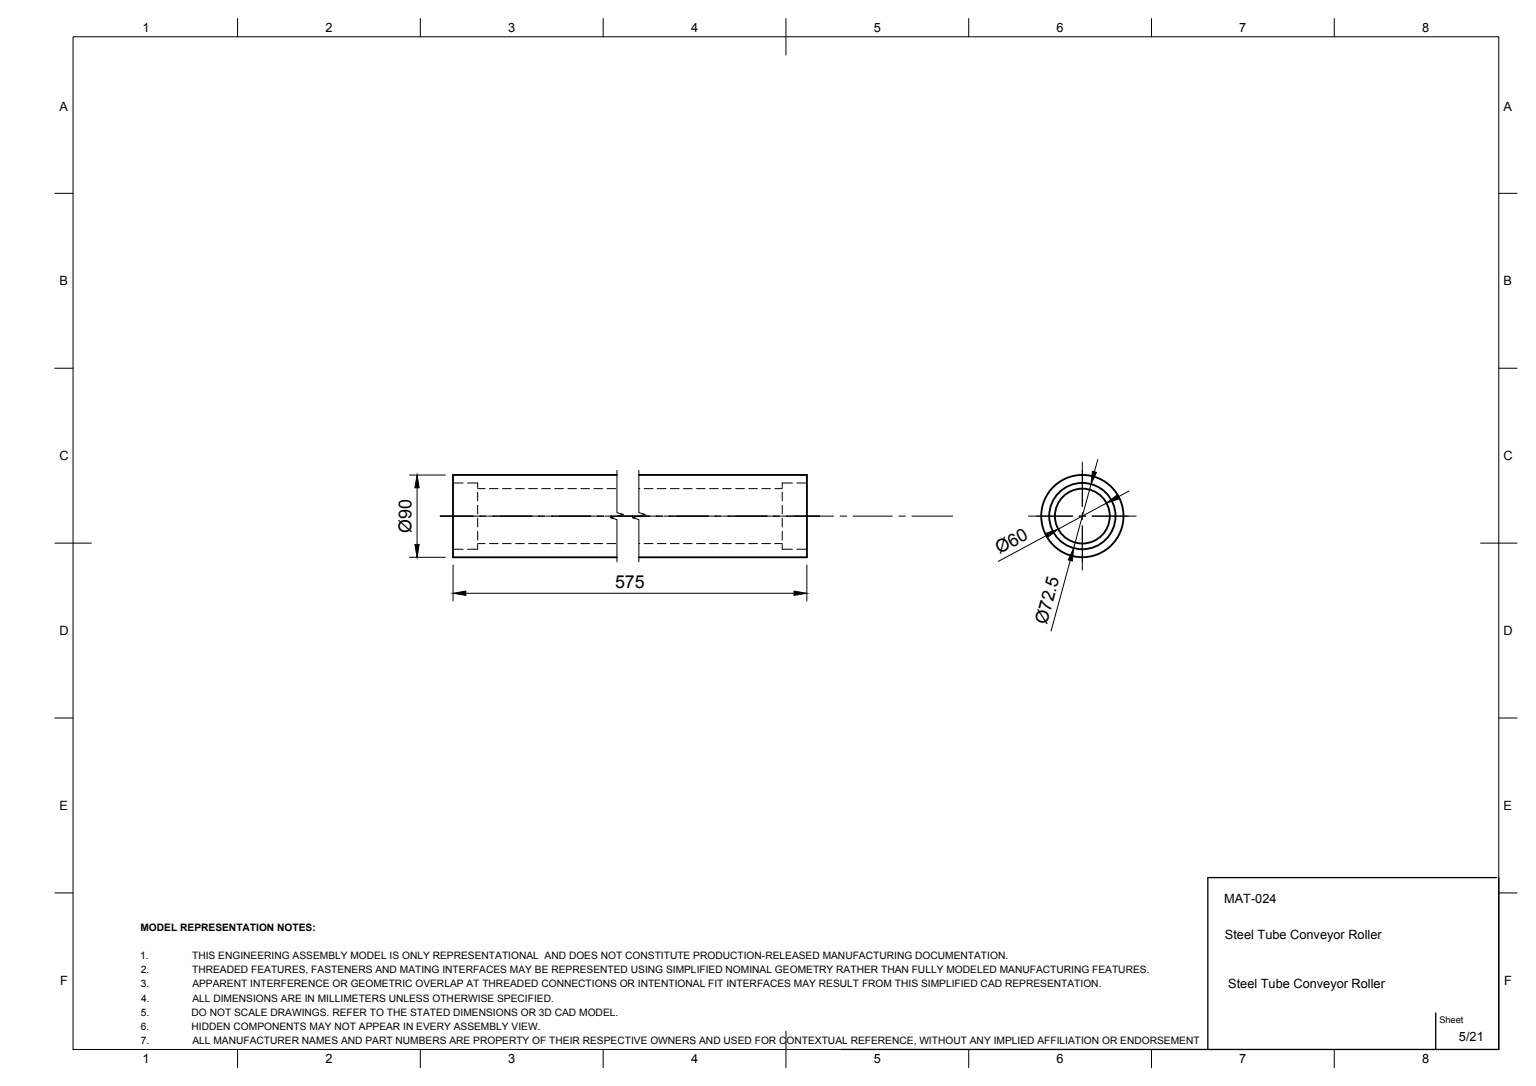
ISO-10303-21;
HEADER;
/* Generated by software containing ST-Developer
 * from STEP Tools, Inc. (www.steptools.com) 
 */

FILE_DESCRIPTION(
/* description */ ('STEP AP214'),
/* implementation_level */ '2;1');

FILE_NAME(
/* name */ 'Steel Tube Conveyor Roller.step',
/* time_stamp */ '2026-11-14T06:34:07-08:00',
/* author */ (''),
/* organization */ (''),
/* preprocessor_version */ 'ST-DEVELOPER v20.2',
/* originating_system */ 'Autodesk Translation Framework v15.17.0.0',
/* authorisation */ '');

FILE_SCHEMA (('AUTOMOTIVE_DESIGN { 1 0 10303 214 3 1 1 }'));
ENDSEC;

DATA;
#10=MECHANICAL_DESIGN_GEOMETRIC_PRESENTATION_REPRESENTATION('',(#7286),#310623);
#7229=SHAPE_REPRESENTATION_RELATIONSHIP('SRR','None',#310902,#7246);
#7246=ADVANCED_BREP_SHAPE_REPRESENTATION('',(#7354),#310611);
#7286=STYLED_ITEM('',(#311003),#7354);
#7354=MANIFOLD_SOLID_BREP('Body1',#93736);
#7638=FACE_BOUND('',#19943,.T.);
#7639=FACE_BOUND('',#19945,.T.);
#7640=FACE_BOUND('',#19947,.T.);
#7641=FACE_BOUND('',#19949,.T.);
#8549=PLANE('',#104125);
#8550=PLANE('',#104126);
#8551=PLANE('',#104127);
#8552=PLANE('',#104128);
#13952=FACE_OUTER_BOUND('',#19938,.T.);
#13953=FACE_OUTER_BOUND('',#19939,.T.);
#13954=FACE_OUTER_BOUND('',#19940,.T.);
#13955=FACE_OUTER_BOUND('',#19941,.T.);
#13956=FACE_OUTER_BOUND('',#19942,.T.);
#13957=FACE_OUTER_BOUND('',#19944,.T.);
#13958=FACE_OUTER_BOUND('',#19946,.T.);
#13959=FACE_OUTER_BOUND('',#19948,.T.);
#19938=EDGE_LOOP('',(#83519,#83520,#83521,#83522));
#19939=EDGE_LOOP('',(#83523,#83524,#83525,#83526));
#19940=EDGE_LOOP('',(#83527,#83528,#83529,#83530));
#19941=EDGE_LOOP('',(#83531,#83532,#83533,#83534));
#19942=EDGE_LOOP('',(#83535));
#19943=EDGE_LOOP('',(#83536));
#19944=EDGE_LOOP('',(#83537));
#19945=EDGE_LOOP('',(#83538));
#19946=EDGE_LOOP('',(#83539));
#19947=EDGE_LOOP('',(#83540));
#19948=EDGE_LOOP('',(#83541));
#19949=EDGE_LOOP('',(#83542));
#24431=LINE('',#275301,#28778);
#24432=LINE('',#275307,#28779);
#24433=LINE('',#275313,#28780);
#24434=LINE('',#275319,#28781);
#28778=VECTOR('',#129118,36.25);
#28779=VECTOR('',#129125,36.25);
#28780=VECTOR('',#129132,45.);
#28781=VECTOR('',#129139,30.);
#34879=CIRCLE('',#104114,36.25);
#34880=CIRCLE('',#104115,36.25);
#34881=CIRCLE('',#104117,36.25);
#34882=CIRCLE('',#104118,36.25);
#34883=CIRCLE('',#104120,45.);
#34884=CIRCLE('',#104121,45.);
#34885=CIRCLE('',#104123,30.);
#34886=CIRCLE('',#104124,30.);
#42853=VERTEX_POINT('',#275298);
#42854=VERTEX_POINT('',#275300);
#42855=VERTEX_POINT('',#275304);
#42856=VERTEX_POINT('',#275306);
#42857=VERTEX_POINT('',#275310);
#42858=VERTEX_POINT('',#275312);
#42859=VERTEX_POINT('',#275316);
#42860=VERTEX_POINT('',#275318);
#56539=EDGE_CURVE('',#42853,#42853,#34879,.T.);
#56540=EDGE_CURVE('',#42853,#42854,#24431,.T.);
#56541=EDGE_CURVE('',#42854,#42854,#34880,.T.);
#56542=EDGE_CURVE('',#42855,#42855,#34881,.T.);
#56543=EDGE_CURVE('',#42855,#42856,#24432,.T.);
#56544=EDGE_CURVE('',#42856,#42856,#34882,.T.);
#56545=EDGE_CURVE('',#42857,#42857,#34883,.T.);
#56546=EDGE_CURVE('',#42857,#42858,#24433,.T.);
#56547=EDGE_CURVE('',#42858,#42858,#34884,.T.);
#56548=EDGE_CURVE('',#42859,#42859,#34885,.T.);
#56549=EDGE_CURVE('',#42859,#42860,#24434,.T.);
#56550=EDGE_CURVE('',#42860,#42860,#34886,.T.);
#83519=ORIENTED_EDGE('',*,*,#56539,.T.);
#83520=ORIENTED_EDGE('',*,*,#56540,.T.);
#83521=ORIENTED_EDGE('',*,*,#56541,.F.);
#83522=ORIENTED_EDGE('',*,*,#56540,.F.);
#83523=ORIENTED_EDGE('',*,*,#56542,.F.);
#83524=ORIENTED_EDGE('',*,*,#56543,.T.);
#83525=ORIENTED_EDGE('',*,*,#56544,.T.);
#83526=ORIENTED_EDGE('',*,*,#56543,.F.);
#83527=ORIENTED_EDGE('',*,*,#56545,.T.);
#83528=ORIENTED_EDGE('',*,*,#56546,.T.);
#83529=ORIENTED_EDGE('',*,*,#56547,.F.);
#83530=ORIENTED_EDGE('',*,*,#56546,.F.);
#83531=ORIENTED_EDGE('',*,*,#56548,.T.);
#83532=ORIENTED_EDGE('',*,*,#56549,.T.);
#83533=ORIENTED_EDGE('',*,*,#56550,.T.);
#83534=ORIENTED_EDGE('',*,*,#56549,.F.);
#83535=ORIENTED_EDGE('',*,*,#56547,.T.);
#83536=ORIENTED_EDGE('',*,*,#56544,.F.);
#83537=ORIENTED_EDGE('',*,*,#56545,.F.);
#83538=ORIENTED_EDGE('',*,*,#56541,.T.);
#83539=ORIENTED_EDGE('',*,*,#56542,.T.);
#83540=ORIENTED_EDGE('',*,*,#56548,.F.);
#83541=ORIENTED_EDGE('',*,*,#56539,.F.);
#83542=ORIENTED_EDGE('',*,*,#56550,.F.);
#87775=CYLINDRICAL_SURFACE('',#104113,36.25);
#87776=CYLINDRICAL_SURFACE('',#104116,36.25);
#87777=CYLINDRICAL_SURFACE('',#104119,45.);
#87778=CYLINDRICAL_SURFACE('',#104122,30.);
#93231=ADVANCED_FACE('',(#13952),#87775,.F.);
#93232=ADVANCED_FACE('',(#13953),#87776,.F.);
#93233=ADVANCED_FACE('',(#13954),#87777,.T.);
#93234=ADVANCED_FACE('',(#13955),#87778,.F.);
#93235=ADVANCED_FACE('',(#13956,#7638),#8549,.T.);
#93236=ADVANCED_FACE('',(#13957,#7639),#8550,.F.);
#93237=ADVANCED_FACE('',(#13958,#7640),#8551,.T.);
#93238=ADVANCED_FACE('',(#13959,#7641),#8552,.T.);
#93736=CLOSED_SHELL('',(#93231,#93232,#93233,#93234,#93235,#93236,#93237,
#93238));
#104112=AXIS2_PLACEMENT_3D('',#275296,#129112,#129113);
#104113=AXIS2_PLACEMENT_3D('',#275297,#129114,#129115);
#104114=AXIS2_PLACEMENT_3D('',#275299,#129116,#129117);
#104115=AXIS2_PLACEMENT_3D('',#275302,#129119,#129120);
#104116=AXIS2_PLACEMENT_3D('',#275303,#129121,#129122);
#104117=AXIS2_PLACEMENT_3D('',#275305,#129123,#129124);
#104118=AXIS2_PLACEMENT_3D('',#275308,#129126,#129127);
#104119=AXIS2_PLACEMENT_3D('',#275309,#129128,#129129);
#104120=AXIS2_PLACEMENT_3D('',#275311,#129130,#129131);
#104121=AXIS2_PLACEMENT_3D('',#275314,#129133,#129134);
#104122=AXIS2_PLACEMENT_3D('',#275315,#129135,#129136);
#104123=AXIS2_PLACEMENT_3D('',#275317,#129137,#129138);
#104124=AXIS2_PLACEMENT_3D('',#275320,#129140,#129141);
#104125=AXIS2_PLACEMENT_3D('',#275321,#129142,#129143);
#104126=AXIS2_PLACEMENT_3D('',#275322,#129144,#129145);
#104127=AXIS2_PLACEMENT_3D('',#275323,#129146,#129147);
#104128=AXIS2_PLACEMENT_3D('',#275324,#129148,#129149);
#129112=DIRECTION('axis',(0.,0.,1.));
#129113=DIRECTION('refdir',(1.,0.,0.));
#129114=DIRECTION('center_axis',(0.,0.,-1.));
#129115=DIRECTION('ref_axis',(-1.,0.,0.));
#129116=DIRECTION('center_axis',(0.,0.,1.));
#129117=DIRECTION('ref_axis',(1.,0.,0.));
#129118=DIRECTION('',(0.,0.,-1.));
#129119=DIRECTION('center_axis',(0.,0.,1.));
#129120=DIRECTION('ref_axis',(1.,0.,0.));
#129121=DIRECTION('center_axis',(0.,0.,1.));
#129122=DIRECTION('ref_axis',(1.,0.,0.));
#129123=DIRECTION('center_axis',(0.,0.,1.));
#129124=DIRECTION('ref_axis',(1.,0.,0.));
#129125=DIRECTION('',(0.,0.,1.));
#129126=DIRECTION('center_axis',(0.,0.,1.));
#129127=DIRECTION('ref_axis',(1.,0.,0.));
#129128=DIRECTION('center_axis',(0.,0.,-1.));
#129129=DIRECTION('ref_axis',(-1.,0.,0.));
#129130=DIRECTION('center_axis',(0.,0.,1.));
#129131=DIRECTION('ref_axis',(1.,0.,0.));
#129132=DIRECTION('',(0.,0.,1.));
#129133=DIRECTION('center_axis',(0.,0.,1.));
#129134=DIRECTION('ref_axis',(1.,0.,0.));
#129135=DIRECTION('center_axis',(0.,0.,-1.));
#129136=DIRECTION('ref_axis',(-1.,0.,0.));
#129137=DIRECTION('center_axis',(0.,0.,1.));
#129138=DIRECTION('ref_axis',(1.,0.,0.));
#129139=DIRECTION('',(0.,0.,-1.));
#129140=DIRECTION('center_axis',(0.,0.,-1.));
#129141=DIRECTION('ref_axis',(-1.,0.,0.));
#129142=DIRECTION('center_axis',(0.,0.,1.));
#129143=DIRECTION('ref_axis',(1.,0.,0.));
#129144=DIRECTION('center_axis',(0.,0.,1.));
#129145=DIRECTION('ref_axis',(1.,0.,0.));
#129146=DIRECTION('center_axis',(0.,0.,1.));
#129147=DIRECTION('ref_axis',(1.,0.,0.));
#129148=DIRECTION('center_axis',(0.,0.,-1.));
#129149=DIRECTION('ref_axis',(1.,0.,0.));
#275296=CARTESIAN_POINT('',(0.,0.,0.));
#275297=CARTESIAN_POINT('Origin',(0.,0.,-260.5));
#275298=CARTESIAN_POINT('',(36.25,-4.43934464690916E-15,-260.5));
#275299=CARTESIAN_POINT('Origin',(0.,0.,-260.5));
#275300=CARTESIAN_POINT('',(36.25,-4.43934464690916E-15,-287.5));
#275301=CARTESIAN_POINT('',(36.25,-4.43934464690916E-15,-260.5));
#275302=CARTESIAN_POINT('Origin',(0.,0.,-287.5));
#275303=CARTESIAN_POINT('Origin',(0.,0.,260.5));
#275304=CARTESIAN_POINT('',(-36.25,-4.43934464690916E-15,260.5));
#275305=CARTESIAN_POINT('Origin',(0.,0.,260.5));
#275306=CARTESIAN_POINT('',(-36.25,-4.43934464690916E-15,287.5));
#275307=CARTESIAN_POINT('',(-36.25,-4.43934464690916E-15,260.5));
#275308=CARTESIAN_POINT('Origin',(0.,0.,287.5));
#275309=CARTESIAN_POINT('Origin',(0.,0.,287.5));
#275310=CARTESIAN_POINT('',(45.,-5.51091059616309E-15,-287.5));
#275311=CARTESIAN_POINT('Origin',(0.,0.,-287.5));
#275312=CARTESIAN_POINT('',(45.,-5.51091059616309E-15,287.5));
#275313=CARTESIAN_POINT('',(45.,-5.51091059616309E-15,287.5));
#275314=CARTESIAN_POINT('Origin',(0.,0.,287.5));
#275315=CARTESIAN_POINT('Origin',(0.,0.,287.5));
#275316=CARTESIAN_POINT('',(30.,-3.67394039744206E-15,260.5));
#275317=CARTESIAN_POINT('Origin',(0.,0.,260.5));
#275318=CARTESIAN_POINT('',(30.,-3.67394039744206E-15,-260.5));
#275319=CARTESIAN_POINT('',(30.,-3.67394039744206E-15,287.5));
#275320=CARTESIAN_POINT('Origin',(0.,0.,-260.5));
#275321=CARTESIAN_POINT('Origin',(0.,0.,287.5));
#275322=CARTESIAN_POINT('Origin',(0.,0.,-287.5));
#275323=CARTESIAN_POINT('Origin',(0.,0.,260.5));
#275324=CARTESIAN_POINT('Origin',(0.,0.,-260.5));
#310589=UNCERTAINTY_MEASURE_WITH_UNIT(LENGTH_MEASURE(0.01),#310624,
'DISTANCE_ACCURACY_VALUE',
'Maximum model space distance between geometric entities at asserted c
onnectivities');
#310601=UNCERTAINTY_MEASURE_WITH_UNIT(LENGTH_MEASURE(0.01),#310624,
'DISTANCE_ACCURACY_VALUE',
'Maximum model space distance between geometric entities at asserted c
onnectivities');
#310611=(
GEOMETRIC_REPRESENTATION_CONTEXT(3)
GLOBAL_UNCERTAINTY_ASSIGNED_CONTEXT((#310589))
GLOBAL_UNIT_ASSIGNED_CONTEXT((#310624,#310626,#310627))
REPRESENTATION_CONTEXT('','3D')
);
#310623=(
GEOMETRIC_REPRESENTATION_CONTEXT(3)
GLOBAL_UNCERTAINTY_ASSIGNED_CONTEXT((#310601))
GLOBAL_UNIT_ASSIGNED_CONTEXT((#310624,#310626,#310627))
REPRESENTATION_CONTEXT('','3D')
);
#310624=(
LENGTH_UNIT()
NAMED_UNIT(*)
SI_UNIT(.MILLI.,.METRE.)
);
#310626=(
NAMED_UNIT(*)
PLANE_ANGLE_UNIT()
SI_UNIT($,.RADIAN.)
);
#310627=(
NAMED_UNIT(*)
SI_UNIT($,.STERADIAN.)
SOLID_ANGLE_UNIT()
);
#310637=SHAPE_DEFINITION_REPRESENTATION(#310796,#310902);
#310796=PRODUCT_DEFINITION_SHAPE('',$,#310924);
#310902=SHAPE_REPRESENTATION('',(#104112),#310611);
#310914=PRODUCT_DEFINITION_CONTEXT('part definition',#310979,'design');
#310924=PRODUCT_DEFINITION('Steel Tube Conveyor Roller',
'Steel Tube Conveyor Roller',#310945,#310914);
#310945=PRODUCT_DEFINITION_FORMATION('',$,#310990);
#310979=APPLICATION_CONTEXT(
'Core Data for Automotive Mechanical Design Process');
#310980=PRODUCT_CONTEXT('part definition',#310979,'mechanical');
#310990=PRODUCT('Steel Tube Conveyor Roller',
'Steel Tube Conveyor Roller',$,(#310980));
#311003=PRESENTATION_STYLE_ASSIGNMENT((#311010));
#311010=SURFACE_STYLE_USAGE(.BOTH.,#311017);
#311017=SURFACE_SIDE_STYLE('',(#311024));
#311024=SURFACE_STYLE_FILL_AREA(#311031);
#311031=FILL_AREA_STYLE('Opaque(97,158,199)',(#311038));
#311038=FILL_AREA_STYLE_COLOUR('Opaque(97,158,199)',#311045);
#311045=COLOUR_RGB('Opaque(97,158,199)',0.380392156862745,0.619607843137255,
0.780392156862745);
ENDSEC;
END-ISO-10303-21;
